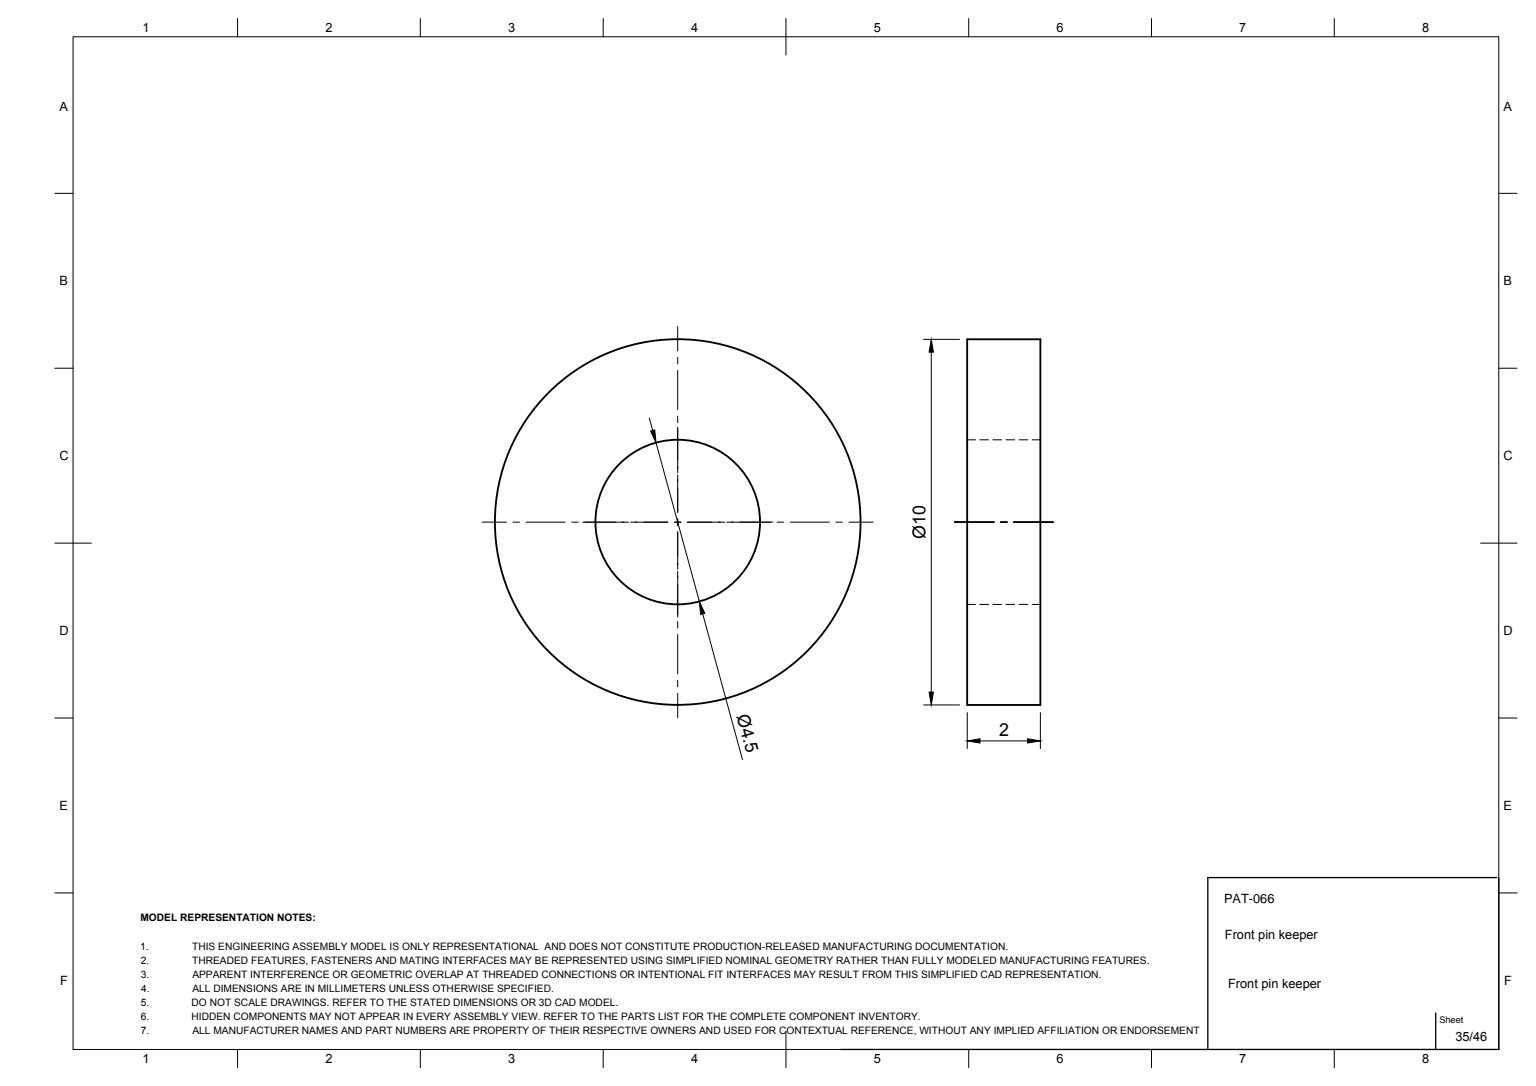
ISO-10303-21;
HEADER;
/* Generated by software containing ST-Developer
 * from STEP Tools, Inc. (www.steptools.com) 
 */

FILE_DESCRIPTION(
/* description */ ('Lever-operated bar clamp (toggle)'),
/* implementation_level */ '2;1');

FILE_NAME(
/* name */ 'Front pin keeper.step',
/* time_stamp */ '2026-10-28T03:25:02-07:00',
/* author */ (''),
/* organization */ (''),
/* preprocessor_version */ 'ST-DEVELOPER v20.2',
/* originating_system */ 'Autodesk Translation Framework v15.17.0.0',
/* authorisation */ '');

FILE_SCHEMA (('AUTOMOTIVE_DESIGN { 1 0 10303 214 3 1 1 }'));
ENDSEC;

DATA;
#10=MECHANICAL_DESIGN_GEOMETRIC_PRESENTATION_REPRESENTATION('',(#444),#12413);
#360=SHAPE_REPRESENTATION_RELATIONSHIP('SRR','None',#12602,#398);
#398=ADVANCED_BREP_SHAPE_REPRESENTATION('',(#489),#12399);
#444=STYLED_ITEM('',(#12869),#489);
#489=MANIFOLD_SOLID_BREP('Body1',#6605);
#629=FACE_BOUND('',#1720,.T.);
#630=FACE_BOUND('',#1722,.T.);
#812=PLANE('',#7652);
#813=PLANE('',#7653);
#1182=FACE_OUTER_BOUND('',#1717,.T.);
#1183=FACE_OUTER_BOUND('',#1718,.T.);
#1184=FACE_OUTER_BOUND('',#1719,.T.);
#1185=FACE_OUTER_BOUND('',#1721,.T.);
#1717=EDGE_LOOP('',(#5599,#5600,#5601,#5602));
#1718=EDGE_LOOP('',(#5603,#5604,#5605,#5606));
#1719=EDGE_LOOP('',(#5607));
#1720=EDGE_LOOP('',(#5608));
#1721=EDGE_LOOP('',(#5609));
#1722=EDGE_LOOP('',(#5610));
#2144=LINE('',#11769,#2585);
#2145=LINE('',#11775,#2586);
#2585=VECTOR('',#9405,0.225);
#2586=VECTOR('',#9412,0.5);
#3007=CIRCLE('',#7647,0.225);
#3008=CIRCLE('',#7648,0.225);
#3009=CIRCLE('',#7650,0.5);
#3010=CIRCLE('',#7651,0.5);
#3474=VERTEX_POINT('',#11766);
#3475=VERTEX_POINT('',#11768);
#3476=VERTEX_POINT('',#11772);
#3477=VERTEX_POINT('',#11774);
#4204=EDGE_CURVE('',#3474,#3474,#3007,.T.);
#4205=EDGE_CURVE('',#3474,#3475,#2144,.T.);
#4206=EDGE_CURVE('',#3475,#3475,#3008,.T.);
#4207=EDGE_CURVE('',#3476,#3476,#3009,.T.);
#4208=EDGE_CURVE('',#3476,#3477,#2145,.T.);
#4209=EDGE_CURVE('',#3477,#3477,#3010,.T.);
#5599=ORIENTED_EDGE('',*,*,#4204,.F.);
#5600=ORIENTED_EDGE('',*,*,#4205,.T.);
#5601=ORIENTED_EDGE('',*,*,#4206,.T.);
#5602=ORIENTED_EDGE('',*,*,#4205,.F.);
#5603=ORIENTED_EDGE('',*,*,#4207,.F.);
#5604=ORIENTED_EDGE('',*,*,#4208,.T.);
#5605=ORIENTED_EDGE('',*,*,#4209,.T.);
#5606=ORIENTED_EDGE('',*,*,#4208,.F.);
#5607=ORIENTED_EDGE('',*,*,#4207,.T.);
#5608=ORIENTED_EDGE('',*,*,#4204,.T.);
#5609=ORIENTED_EDGE('',*,*,#4209,.F.);
#5610=ORIENTED_EDGE('',*,*,#4206,.F.);
#6137=CYLINDRICAL_SURFACE('',#7646,0.225);
#6138=CYLINDRICAL_SURFACE('',#7649,0.5);
#6457=ADVANCED_FACE('',(#1182),#6137,.F.);
#6458=ADVANCED_FACE('',(#1183),#6138,.T.);
#6459=ADVANCED_FACE('',(#1184,#629),#812,.T.);
#6460=ADVANCED_FACE('',(#1185,#630),#813,.F.);
#6605=CLOSED_SHELL('',(#6457,#6458,#6459,#6460));
#7645=AXIS2_PLACEMENT_3D('',#11764,#9399,#9400);
#7646=AXIS2_PLACEMENT_3D('',#11765,#9401,#9402);
#7647=AXIS2_PLACEMENT_3D('',#11767,#9403,#9404);
#7648=AXIS2_PLACEMENT_3D('',#11770,#9406,#9407);
#7649=AXIS2_PLACEMENT_3D('',#11771,#9408,#9409);
#7650=AXIS2_PLACEMENT_3D('',#11773,#9410,#9411);
#7651=AXIS2_PLACEMENT_3D('',#11776,#9413,#9414);
#7652=AXIS2_PLACEMENT_3D('',#11777,#9415,#9416);
#7653=AXIS2_PLACEMENT_3D('',#11778,#9417,#9418);
#9399=DIRECTION('axis',(0.,0.,1.));
#9400=DIRECTION('refdir',(1.,0.,0.));
#9401=DIRECTION('center_axis',(0.,1.,0.));
#9402=DIRECTION('ref_axis',(1.,0.,0.));
#9403=DIRECTION('center_axis',(0.,-1.,0.));
#9404=DIRECTION('ref_axis',(1.,0.,0.));
#9405=DIRECTION('',(0.,-1.,0.));
#9406=DIRECTION('center_axis',(0.,-1.,0.));
#9407=DIRECTION('ref_axis',(1.,0.,0.));
#9408=DIRECTION('center_axis',(0.,1.,0.));
#9409=DIRECTION('ref_axis',(1.,0.,0.));
#9410=DIRECTION('center_axis',(0.,1.,0.));
#9411=DIRECTION('ref_axis',(1.,0.,0.));
#9412=DIRECTION('',(0.,-1.,0.));
#9413=DIRECTION('center_axis',(0.,1.,0.));
#9414=DIRECTION('ref_axis',(1.,0.,0.));
#9415=DIRECTION('center_axis',(0.,1.,0.));
#9416=DIRECTION('ref_axis',(1.,0.,0.));
#9417=DIRECTION('center_axis',(0.,1.,0.));
#9418=DIRECTION('ref_axis',(1.,0.,0.));
#11764=CARTESIAN_POINT('',(0.,0.,0.));
#11765=CARTESIAN_POINT('Origin',(-2.82632109303527,-5.9,8.79263101785268));
#11766=CARTESIAN_POINT('',(-3.05132109303527,-5.7,8.79263101785268));
#11767=CARTESIAN_POINT('Origin',(-2.82632109303527,-5.7,8.79263101785268));
#11768=CARTESIAN_POINT('',(-3.05132109303527,-5.9,8.79263101785268));
#11769=CARTESIAN_POINT('',(-3.05132109303527,-5.9,8.79263101785268));
#11770=CARTESIAN_POINT('Origin',(-2.82632109303527,-5.9,8.79263101785268));
#11771=CARTESIAN_POINT('Origin',(-2.82632109303527,-5.9,8.79263101785268));
#11772=CARTESIAN_POINT('',(-3.32632109303527,-5.7,8.79263101785268));
#11773=CARTESIAN_POINT('Origin',(-2.82632109303527,-5.7,8.79263101785268));
#11774=CARTESIAN_POINT('',(-3.32632109303527,-5.9,8.79263101785268));
#11775=CARTESIAN_POINT('',(-3.32632109303527,-5.9,8.79263101785268));
#11776=CARTESIAN_POINT('Origin',(-2.82632109303527,-5.9,8.79263101785268));
#11777=CARTESIAN_POINT('Origin',(-2.82632109303527,-5.7,8.79263101785268));
#11778=CARTESIAN_POINT('Origin',(-2.82632109303527,-5.9,8.79263101785268));
#12353=UNCERTAINTY_MEASURE_WITH_UNIT(LENGTH_MEASURE(0.001),#12414,
'DISTANCE_ACCURACY_VALUE',
'Maximum model space distance between geometric entities at asserted c
onnectivities');
#12367=UNCERTAINTY_MEASURE_WITH_UNIT(LENGTH_MEASURE(0.001),#12414,
'DISTANCE_ACCURACY_VALUE',
'Maximum model space distance between geometric entities at asserted c
onnectivities');
#12399=(
GEOMETRIC_REPRESENTATION_CONTEXT(3)
GLOBAL_UNCERTAINTY_ASSIGNED_CONTEXT((#12353))
GLOBAL_UNIT_ASSIGNED_CONTEXT((#12414,#12416,#12417))
REPRESENTATION_CONTEXT('','3D')
);
#12413=(
GEOMETRIC_REPRESENTATION_CONTEXT(3)
GLOBAL_UNCERTAINTY_ASSIGNED_CONTEXT((#12367))
GLOBAL_UNIT_ASSIGNED_CONTEXT((#12414,#12416,#12417))
REPRESENTATION_CONTEXT('','3D')
);
#12414=(
LENGTH_UNIT()
NAMED_UNIT(*)
SI_UNIT(.CENTI.,.METRE.)
);
#12416=(
NAMED_UNIT(*)
PLANE_ANGLE_UNIT()
SI_UNIT($,.RADIAN.)
);
#12417=(
NAMED_UNIT(*)
SI_UNIT($,.STERADIAN.)
SOLID_ANGLE_UNIT()
);
#12449=SHAPE_DEFINITION_REPRESENTATION(#12501,#12602);
#12501=PRODUCT_DEFINITION_SHAPE('',$,#12648);
#12602=SHAPE_REPRESENTATION('',(#7645),#12399);
#12616=PRODUCT_DEFINITION_CONTEXT('part definition',#12753,'design');
#12648=PRODUCT_DEFINITION('Front pin keeper','Front pin keeper',#12693,
#12616);
#12693=PRODUCT_DEFINITION_FORMATION('',$,#12786);
#12753=APPLICATION_CONTEXT(
'Core Data for Automotive Mechanical Design Process');
#12754=PRODUCT_CONTEXT('part definition',#12753,'mechanical');
#12786=PRODUCT('Front pin keeper','Front pin keeper','Front pin keeper',
(#12754));
#12863=COLOUR_RGB('Grey',0.48,0.52,0.57);
#12864=FILL_AREA_STYLE_COLOUR('',#12863);
#12865=FILL_AREA_STYLE('',(#12864));
#12866=SURFACE_STYLE_FILL_AREA(#12865);
#12867=SURFACE_SIDE_STYLE('',(#12866));
#12868=SURFACE_STYLE_USAGE(.BOTH.,#12867);
#12869=PRESENTATION_STYLE_ASSIGNMENT((#12868));
ENDSEC;
END-ISO-10303-21;
